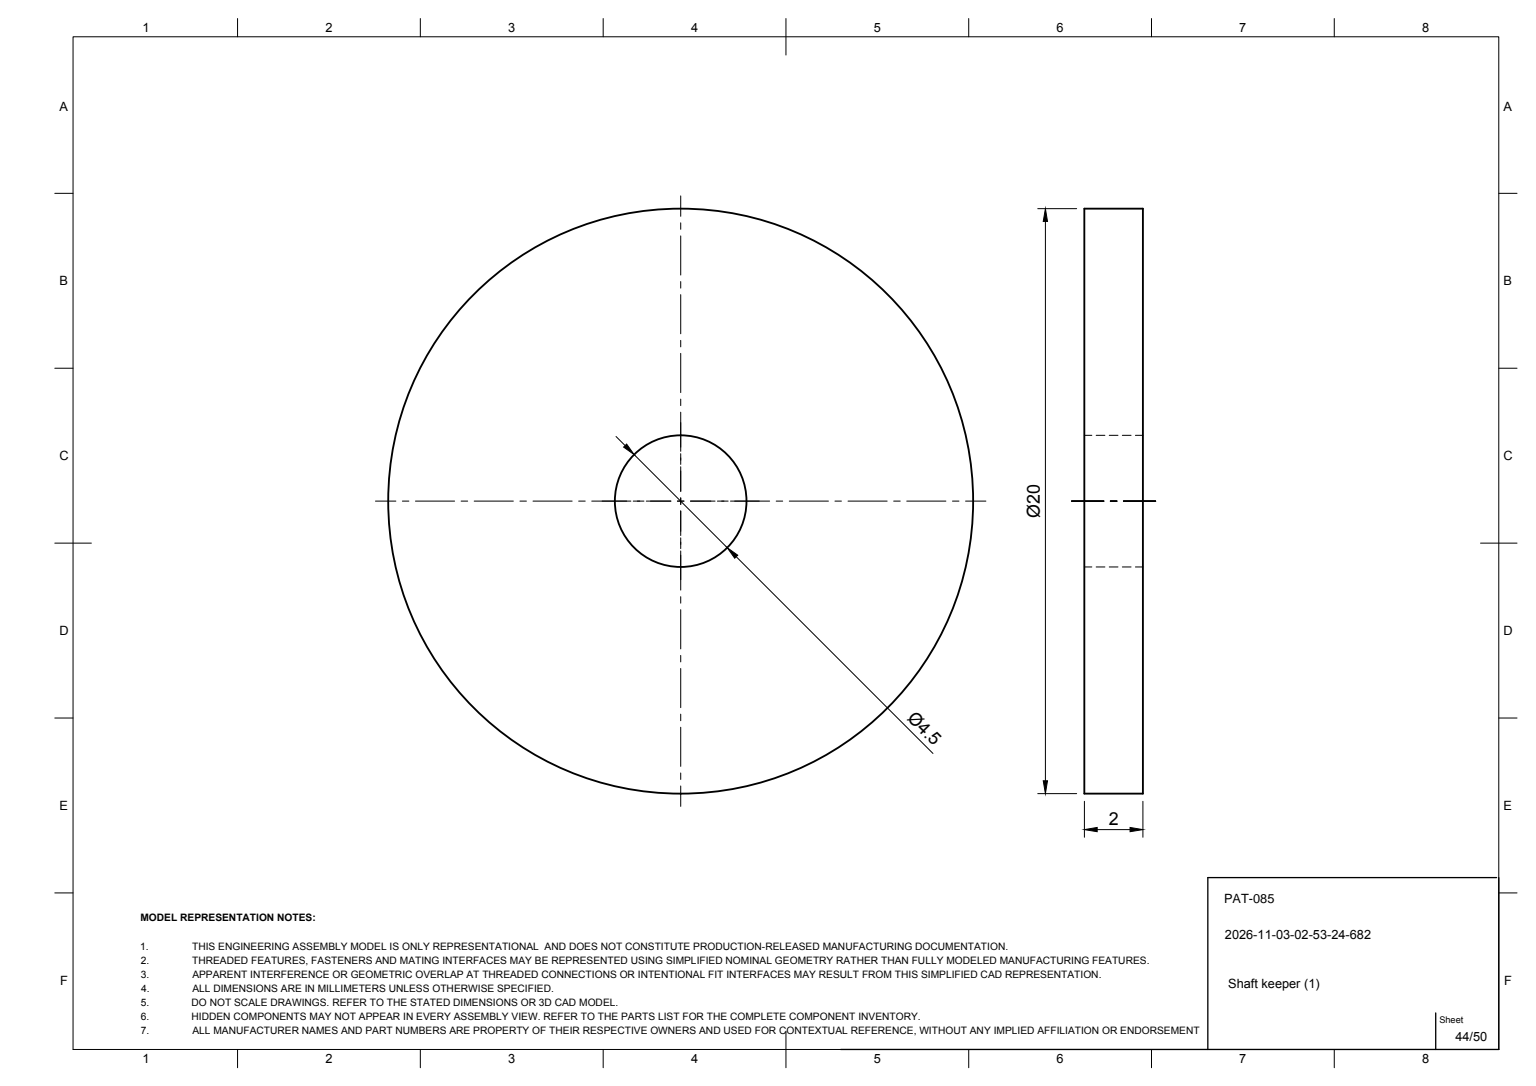
ISO-10303-21;
HEADER;
/* Generated by software containing ST-Developer
 * from STEP Tools, Inc. (www.steptools.com) 
 */

FILE_DESCRIPTION(
/* description */ ('Rack and pinion manual slide'),
/* implementation_level */ '2;1');

FILE_NAME(
/* name */ 'Shaft keeper (1).step',
/* time_stamp */ '2026-10-28T03:22:49-07:00',
/* author */ (''),
/* organization */ (''),
/* preprocessor_version */ 'ST-DEVELOPER v20.2',
/* originating_system */ 'Autodesk Translation Framework v15.17.0.0',
/* authorisation */ '');

FILE_SCHEMA (('AUTOMOTIVE_DESIGN { 1 0 10303 214 3 1 1 }'));
ENDSEC;

DATA;
#10=MECHANICAL_DESIGN_GEOMETRIC_PRESENTATION_REPRESENTATION('',(#775),#34851);
#676=SHAPE_REPRESENTATION_RELATIONSHIP('SRR','None',#35115,#722);
#722=ADVANCED_BREP_SHAPE_REPRESENTATION('',(#825),#34840);
#775=STYLED_ITEM('',(#35411),#825);
#825=MANIFOLD_SOLID_BREP('Body1',#13798);
#1024=FACE_BOUND('',#3042,.T.);
#1025=FACE_BOUND('',#3044,.T.);
#1458=PLANE('',#15278);
#1459=PLANE('',#15279);
#2109=FACE_OUTER_BOUND('',#3039,.T.);
#2110=FACE_OUTER_BOUND('',#3040,.T.);
#2111=FACE_OUTER_BOUND('',#3041,.T.);
#2112=FACE_OUTER_BOUND('',#3043,.T.);
#3039=EDGE_LOOP('',(#12038,#12039,#12040,#12041));
#3040=EDGE_LOOP('',(#12042,#12043,#12044,#12045));
#3041=EDGE_LOOP('',(#12046));
#3042=EDGE_LOOP('',(#12047));
#3043=EDGE_LOOP('',(#12048));
#3044=EDGE_LOOP('',(#12049));
#4282=LINE('',#22721,#5573);
#4283=LINE('',#22727,#5574);
#5573=VECTOR('',#18572,0.225);
#5574=VECTOR('',#18579,1.);
#6134=CIRCLE('',#15273,0.225);
#6135=CIRCLE('',#15274,0.225);
#6136=CIRCLE('',#15276,1.);
#6137=CIRCLE('',#15277,1.);
#7163=VERTEX_POINT('',#22718);
#7164=VERTEX_POINT('',#22720);
#7165=VERTEX_POINT('',#22724);
#7166=VERTEX_POINT('',#22726);
#8831=EDGE_CURVE('',#7163,#7163,#6134,.T.);
#8832=EDGE_CURVE('',#7163,#7164,#4282,.T.);
#8833=EDGE_CURVE('',#7164,#7164,#6135,.T.);
#8834=EDGE_CURVE('',#7165,#7165,#6136,.T.);
#8835=EDGE_CURVE('',#7165,#7166,#4283,.T.);
#8836=EDGE_CURVE('',#7166,#7166,#6137,.T.);
#12038=ORIENTED_EDGE('',*,*,#8831,.F.);
#12039=ORIENTED_EDGE('',*,*,#8832,.T.);
#12040=ORIENTED_EDGE('',*,*,#8833,.T.);
#12041=ORIENTED_EDGE('',*,*,#8832,.F.);
#12042=ORIENTED_EDGE('',*,*,#8834,.F.);
#12043=ORIENTED_EDGE('',*,*,#8835,.T.);
#12044=ORIENTED_EDGE('',*,*,#8836,.T.);
#12045=ORIENTED_EDGE('',*,*,#8835,.F.);
#12046=ORIENTED_EDGE('',*,*,#8834,.T.);
#12047=ORIENTED_EDGE('',*,*,#8831,.T.);
#12048=ORIENTED_EDGE('',*,*,#8836,.F.);
#12049=ORIENTED_EDGE('',*,*,#8833,.F.);
#12973=CYLINDRICAL_SURFACE('',#15272,0.225);
#12974=CYLINDRICAL_SURFACE('',#15275,1.);
#13587=ADVANCED_FACE('',(#2109),#12973,.F.);
#13588=ADVANCED_FACE('',(#2110),#12974,.T.);
#13589=ADVANCED_FACE('',(#2111,#1024),#1458,.T.);
#13590=ADVANCED_FACE('',(#2112,#1025),#1459,.F.);
#13798=CLOSED_SHELL('',(#13587,#13588,#13589,#13590));
#15271=AXIS2_PLACEMENT_3D('',#22716,#18566,#18567);
#15272=AXIS2_PLACEMENT_3D('',#22717,#18568,#18569);
#15273=AXIS2_PLACEMENT_3D('',#22719,#18570,#18571);
#15274=AXIS2_PLACEMENT_3D('',#22722,#18573,#18574);
#15275=AXIS2_PLACEMENT_3D('',#22723,#18575,#18576);
#15276=AXIS2_PLACEMENT_3D('',#22725,#18577,#18578);
#15277=AXIS2_PLACEMENT_3D('',#22728,#18580,#18581);
#15278=AXIS2_PLACEMENT_3D('',#22729,#18582,#18583);
#15279=AXIS2_PLACEMENT_3D('',#22730,#18584,#18585);
#18566=DIRECTION('axis',(0.,0.,1.));
#18567=DIRECTION('refdir',(1.,0.,0.));
#18568=DIRECTION('center_axis',(0.,1.,0.));
#18569=DIRECTION('ref_axis',(1.,0.,0.));
#18570=DIRECTION('center_axis',(0.,-1.,0.));
#18571=DIRECTION('ref_axis',(1.,0.,0.));
#18572=DIRECTION('',(0.,-1.,0.));
#18573=DIRECTION('center_axis',(0.,-1.,0.));
#18574=DIRECTION('ref_axis',(1.,0.,0.));
#18575=DIRECTION('center_axis',(0.,1.,0.));
#18576=DIRECTION('ref_axis',(1.,0.,0.));
#18577=DIRECTION('center_axis',(0.,1.,0.));
#18578=DIRECTION('ref_axis',(1.,0.,0.));
#18579=DIRECTION('',(0.,-1.,0.));
#18580=DIRECTION('center_axis',(0.,1.,0.));
#18581=DIRECTION('ref_axis',(1.,0.,0.));
#18582=DIRECTION('center_axis',(0.,1.,0.));
#18583=DIRECTION('ref_axis',(1.,0.,0.));
#18584=DIRECTION('center_axis',(0.,1.,0.));
#18585=DIRECTION('ref_axis',(1.,0.,0.));
#22716=CARTESIAN_POINT('',(0.,0.,0.));
#22717=CARTESIAN_POINT('Origin',(11.,7.9,10.25));
#22718=CARTESIAN_POINT('',(10.775,8.1,10.25));
#22719=CARTESIAN_POINT('Origin',(11.,8.1,10.25));
#22720=CARTESIAN_POINT('',(10.775,7.9,10.25));
#22721=CARTESIAN_POINT('',(10.775,7.9,10.25));
#22722=CARTESIAN_POINT('Origin',(11.,7.9,10.25));
#22723=CARTESIAN_POINT('Origin',(11.,7.9,10.25));
#22724=CARTESIAN_POINT('',(10.,8.1,10.25));
#22725=CARTESIAN_POINT('Origin',(11.,8.1,10.25));
#22726=CARTESIAN_POINT('',(10.,7.9,10.25));
#22727=CARTESIAN_POINT('',(10.,7.9,10.25));
#22728=CARTESIAN_POINT('Origin',(11.,7.9,10.25));
#22729=CARTESIAN_POINT('Origin',(11.,8.1,10.25));
#22730=CARTESIAN_POINT('Origin',(11.,7.9,10.25));
#34786=UNCERTAINTY_MEASURE_WITH_UNIT(LENGTH_MEASURE(0.001),#34852,
'DISTANCE_ACCURACY_VALUE',
'Maximum model space distance between geometric entities at asserted c
onnectivities');
#34797=UNCERTAINTY_MEASURE_WITH_UNIT(LENGTH_MEASURE(0.001),#34852,
'DISTANCE_ACCURACY_VALUE',
'Maximum model space distance between geometric entities at asserted c
onnectivities');
#34840=(
GEOMETRIC_REPRESENTATION_CONTEXT(3)
GLOBAL_UNCERTAINTY_ASSIGNED_CONTEXT((#34786))
GLOBAL_UNIT_ASSIGNED_CONTEXT((#34852,#34854,#34855))
REPRESENTATION_CONTEXT('','3D')
);
#34851=(
GEOMETRIC_REPRESENTATION_CONTEXT(3)
GLOBAL_UNCERTAINTY_ASSIGNED_CONTEXT((#34797))
GLOBAL_UNIT_ASSIGNED_CONTEXT((#34852,#34854,#34855))
REPRESENTATION_CONTEXT('','3D')
);
#34852=(
LENGTH_UNIT()
NAMED_UNIT(*)
SI_UNIT(.CENTI.,.METRE.)
);
#34854=(
NAMED_UNIT(*)
PLANE_ANGLE_UNIT()
SI_UNIT($,.RADIAN.)
);
#34855=(
NAMED_UNIT(*)
SI_UNIT($,.STERADIAN.)
SOLID_ANGLE_UNIT()
);
#34898=SHAPE_DEFINITION_REPRESENTATION(#34959,#35115);
#34959=PRODUCT_DEFINITION_SHAPE('',$,#35169);
#35115=SHAPE_REPRESENTATION('',(#15271),#34840);
#35126=PRODUCT_DEFINITION_CONTEXT('part definition',#35287,'design');
#35169=PRODUCT_DEFINITION('Shaft keeper (1)','Shaft keeper (1)',#35222,#35126);
#35222=PRODUCT_DEFINITION_FORMATION('',$,#35331);
#35287=APPLICATION_CONTEXT(
'Core Data for Automotive Mechanical Design Process');
#35288=PRODUCT_CONTEXT('part definition',#35287,'mechanical');
#35331=PRODUCT('Shaft keeper (1)','Shaft keeper (1)','Shaft keeper (1)',(#35288));
#35405=COLOUR_RGB('Grey',0.48,0.52,0.57);
#35406=FILL_AREA_STYLE_COLOUR('',#35405);
#35407=FILL_AREA_STYLE('',(#35406));
#35408=SURFACE_STYLE_FILL_AREA(#35407);
#35409=SURFACE_SIDE_STYLE('',(#35408));
#35410=SURFACE_STYLE_USAGE(.BOTH.,#35409);
#35411=PRESENTATION_STYLE_ASSIGNMENT((#35410));
ENDSEC;
END-ISO-10303-21;
